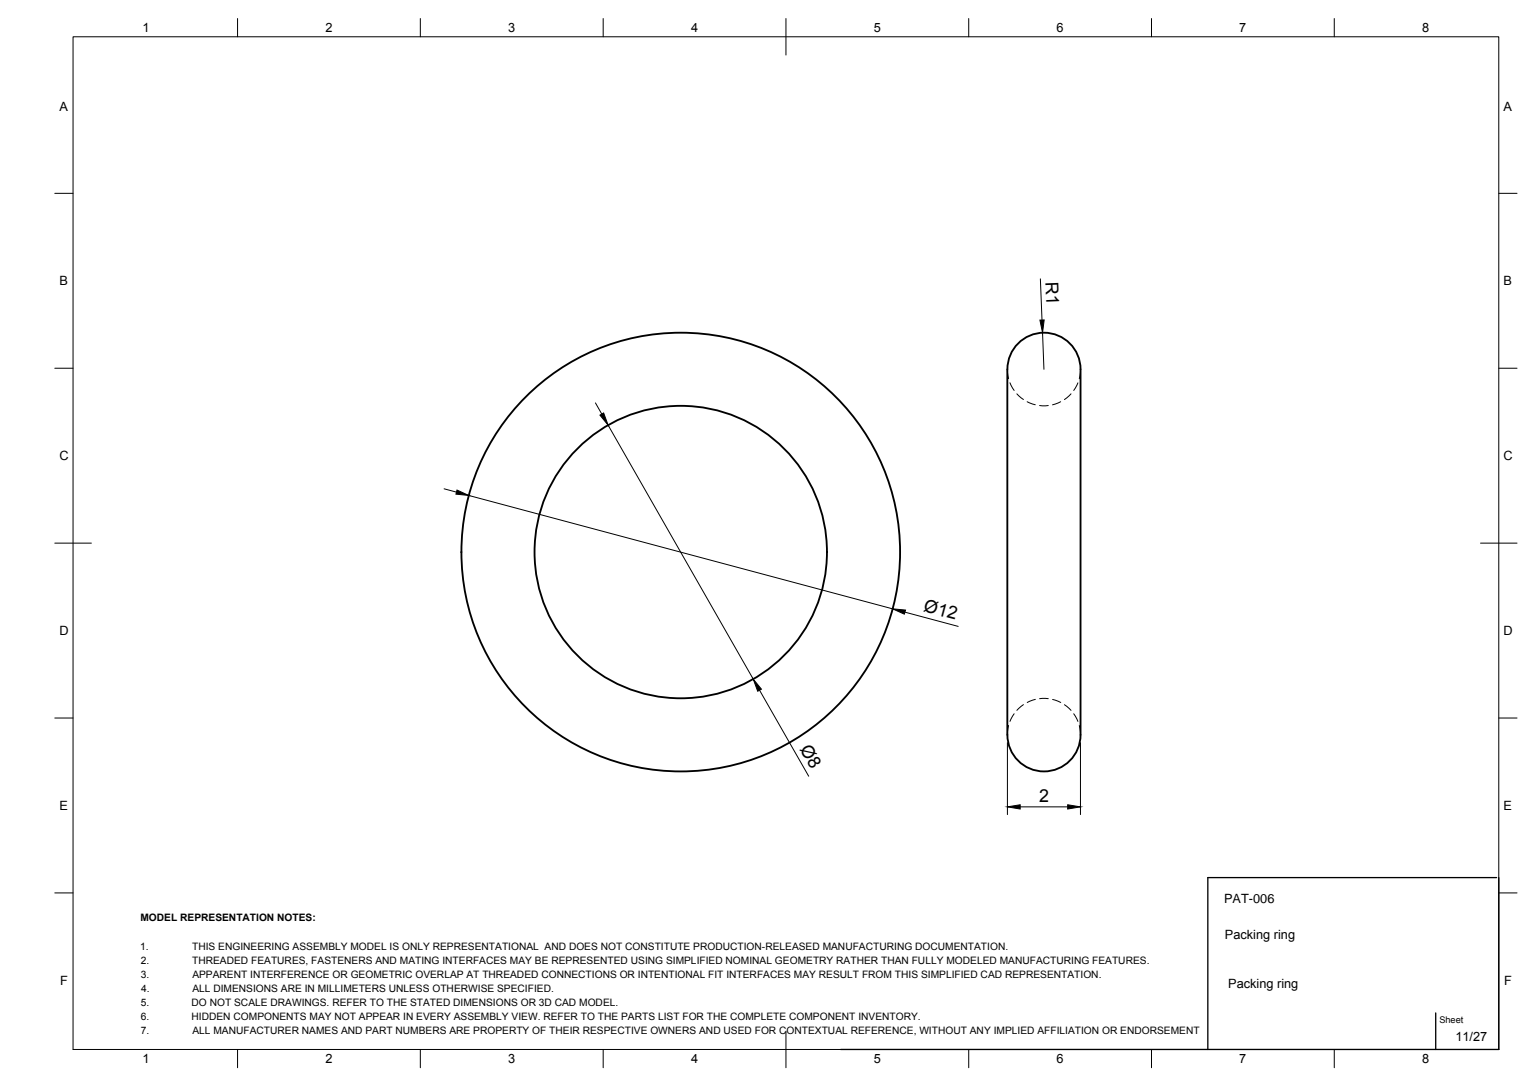
ISO-10303-21;
HEADER;
/* Generated by software containing ST-Developer
 * from STEP Tools, Inc. (www.steptools.com) 
 */

FILE_DESCRIPTION(
/* description */ ('Ball-type isolation valve (generic)'),
/* implementation_level */ '2;1');

FILE_NAME(
/* name */ 'Packing ring.step',
/* time_stamp */ '2026-10-27T10:53:05-07:00',
/* author */ (''),
/* organization */ (''),
/* preprocessor_version */ 'ST-DEVELOPER v20.2',
/* originating_system */ 'Autodesk Translation Framework v15.17.0.0',
/* authorisation */ '');

FILE_SCHEMA (('AUTOMOTIVE_DESIGN { 1 0 10303 214 3 1 1 }'));
ENDSEC;

DATA;
#10=MECHANICAL_DESIGN_GEOMETRIC_PRESENTATION_REPRESENTATION('',(#283),#7425);
#224=TOROIDAL_SURFACE('',#4549,0.5,0.1);
#231=SHAPE_REPRESENTATION_RELATIONSHIP('SRR','None',#7541,#257);
#257=ADVANCED_BREP_SHAPE_REPRESENTATION('',(#309),#7404);
#283=STYLED_ITEM('',(#7737),#309);
#309=MANIFOLD_SOLID_BREP('Body1',#4088);
#653=FACE_OUTER_BOUND('',#947,.T.);
#947=EDGE_LOOP('',(#3089,#3090,#3091,#3092));
#1849=CIRCLE('',#4550,0.1);
#1850=CIRCLE('',#4551,0.4);
#2062=VERTEX_POINT('',#6547);
#2437=EDGE_CURVE('',#2062,#2062,#1849,.T.);
#2438=EDGE_CURVE('',#2062,#2062,#1850,.T.);
#3089=ORIENTED_EDGE('',*,*,#2437,.F.);
#3090=ORIENTED_EDGE('',*,*,#2438,.T.);
#3091=ORIENTED_EDGE('',*,*,#2437,.T.);
#3092=ORIENTED_EDGE('',*,*,#2438,.F.);
#3907=ADVANCED_FACE('',(#653),#224,.T.);
#4088=CLOSED_SHELL('',(#3907));
#4548=AXIS2_PLACEMENT_3D('',#6545,#5285,#5286);
#4549=AXIS2_PLACEMENT_3D('',#6546,#5287,#5288);
#4550=AXIS2_PLACEMENT_3D('',#6548,#5289,#5290);
#4551=AXIS2_PLACEMENT_3D('',#6549,#5291,#5292);
#5285=DIRECTION('axis',(0.,0.,1.));
#5286=DIRECTION('refdir',(1.,0.,0.));
#5287=DIRECTION('center_axis',(0.,0.,1.));
#5288=DIRECTION('ref_axis',(1.,0.,0.));
#5289=DIRECTION('center_axis',(1.22464679914735E-16,-1.,0.));
#5290=DIRECTION('ref_axis',(-1.,-1.22464679914735E-16,0.));
#5291=DIRECTION('center_axis',(0.,0.,-1.));
#5292=DIRECTION('ref_axis',(1.,0.,0.));
#6545=CARTESIAN_POINT('',(0.,0.,0.));
#6546=CARTESIAN_POINT('Origin',(0.,0.,8.1));
#6547=CARTESIAN_POINT('',(-0.4,-4.89858719658941E-17,8.1));
#6548=CARTESIAN_POINT('Origin',(-0.5,-6.12323399573677E-17,8.1));
#6549=CARTESIAN_POINT('Origin',(0.,0.,8.1));
#7374=UNCERTAINTY_MEASURE_WITH_UNIT(LENGTH_MEASURE(0.001),#7426,
'DISTANCE_ACCURACY_VALUE',
'Maximum model space distance between geometric entities at asserted c
onnectivities');
#7395=UNCERTAINTY_MEASURE_WITH_UNIT(LENGTH_MEASURE(0.001),#7426,
'DISTANCE_ACCURACY_VALUE',
'Maximum model space distance between geometric entities at asserted c
onnectivities');
#7404=(
GEOMETRIC_REPRESENTATION_CONTEXT(3)
GLOBAL_UNCERTAINTY_ASSIGNED_CONTEXT((#7374))
GLOBAL_UNIT_ASSIGNED_CONTEXT((#7426,#7428,#7429))
REPRESENTATION_CONTEXT('','3D')
);
#7425=(
GEOMETRIC_REPRESENTATION_CONTEXT(3)
GLOBAL_UNCERTAINTY_ASSIGNED_CONTEXT((#7395))
GLOBAL_UNIT_ASSIGNED_CONTEXT((#7426,#7428,#7429))
REPRESENTATION_CONTEXT('','3D')
);
#7426=(
LENGTH_UNIT()
NAMED_UNIT(*)
SI_UNIT(.CENTI.,.METRE.)
);
#7428=(
NAMED_UNIT(*)
PLANE_ANGLE_UNIT()
SI_UNIT($,.RADIAN.)
);
#7429=(
NAMED_UNIT(*)
SI_UNIT($,.STERADIAN.)
SOLID_ANGLE_UNIT()
);
#7438=SHAPE_DEFINITION_REPRESENTATION(#7467,#7541);
#7467=PRODUCT_DEFINITION_SHAPE('',$,#7571);
#7541=SHAPE_REPRESENTATION('',(#4548),#7404);
#7562=PRODUCT_DEFINITION_CONTEXT('part definition',#7651,'design');
#7571=PRODUCT_DEFINITION('Packing ring','Packing ring',#7600,#7562);
#7600=PRODUCT_DEFINITION_FORMATION('',$,#7661);
#7651=APPLICATION_CONTEXT(
'Core Data for Automotive Mechanical Design Process');
#7652=PRODUCT_CONTEXT('part definition',#7651,'mechanical');
#7661=PRODUCT('Packing ring','Packing ring','Packing ring',(#7652));
#7731=COLOUR_RGB('Sky Blue',0.24,0.69,0.87);
#7732=FILL_AREA_STYLE_COLOUR('',#7731);
#7733=FILL_AREA_STYLE('',(#7732));
#7734=SURFACE_STYLE_FILL_AREA(#7733);
#7735=SURFACE_SIDE_STYLE('',(#7734));
#7736=SURFACE_STYLE_USAGE(.BOTH.,#7735);
#7737=PRESENTATION_STYLE_ASSIGNMENT((#7736));
ENDSEC;
END-ISO-10303-21;
